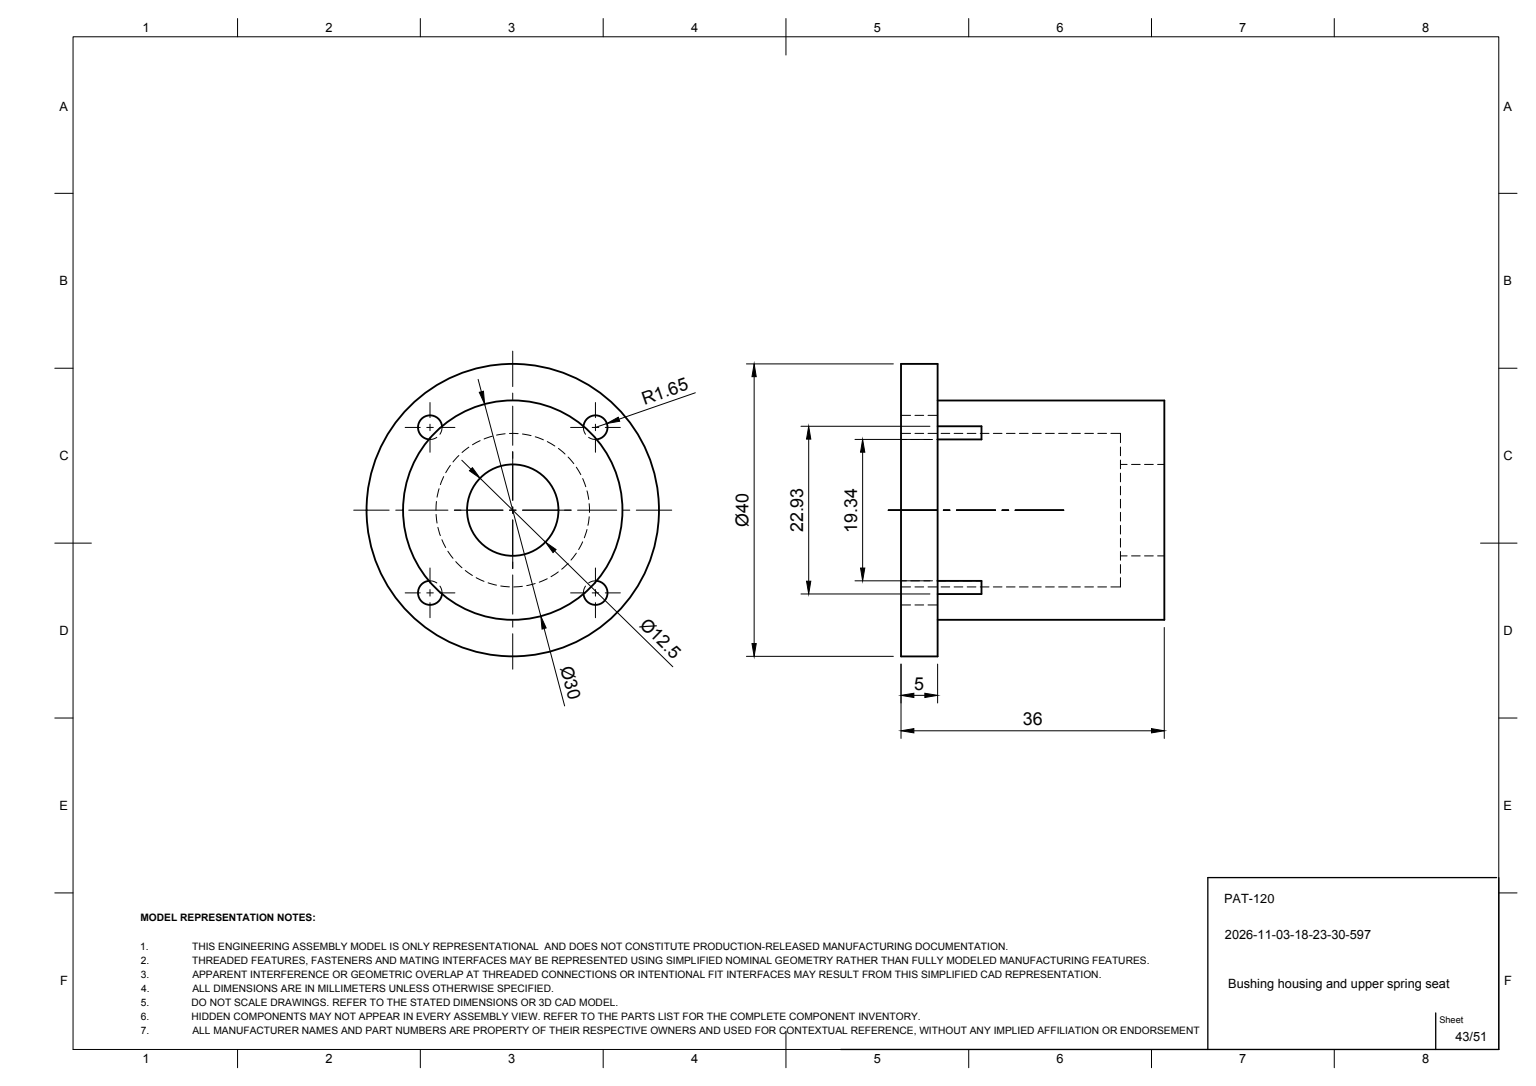
ISO-10303-21;
HEADER;
/* Generated by software containing ST-Developer
 * from STEP Tools, Inc. (www.steptools.com) 
 */

FILE_DESCRIPTION(
/* description */ ('Vibration shaker table dummy'),
/* implementation_level */ '2;1');

FILE_NAME(
/* name */ 'Bushing housing and upper spring seat.step',
/* time_stamp */ '2026-10-27T10:55:14-07:00',
/* author */ (''),
/* organization */ (''),
/* preprocessor_version */ 'ST-DEVELOPER v20.2',
/* originating_system */ 'Autodesk Translation Framework v15.17.0.0',
/* authorisation */ '');

FILE_SCHEMA (('AUTOMOTIVE_DESIGN { 1 0 10303 214 3 1 1 }'));
ENDSEC;

DATA;
#10=MECHANICAL_DESIGN_GEOMETRIC_PRESENTATION_REPRESENTATION('',(#724),#22394);
#632=SHAPE_REPRESENTATION_RELATIONSHIP('SRR','None',#22679,#678);
#678=ADVANCED_BREP_SHAPE_REPRESENTATION('',(#768),#22385);
#724=STYLED_ITEM('',(#22961),#768);
#768=MANIFOLD_SOLID_BREP('Body1',#9244);
#1007=FACE_BOUND('',#2465,.T.);
#1008=FACE_BOUND('',#2467,.T.);
#1009=FACE_BOUND('',#2471,.T.);
#1010=FACE_BOUND('',#2472,.T.);
#1011=FACE_BOUND('',#2473,.T.);
#1012=FACE_BOUND('',#2474,.T.);
#1013=FACE_BOUND('',#2475,.T.);
#1014=FACE_BOUND('',#2477,.T.);
#1278=PLANE('',#10518);
#1279=PLANE('',#10525);
#1280=PLANE('',#10532);
#1281=PLANE('',#10539);
#1282=PLANE('',#10556);
#1283=PLANE('',#10558);
#1284=PLANE('',#10564);
#1285=PLANE('',#10565);
#1724=FACE_OUTER_BOUND('',#2454,.T.);
#1725=FACE_OUTER_BOUND('',#2455,.T.);
#1726=FACE_OUTER_BOUND('',#2456,.T.);
#1727=FACE_OUTER_BOUND('',#2457,.T.);
#1728=FACE_OUTER_BOUND('',#2458,.T.);
#1729=FACE_OUTER_BOUND('',#2459,.T.);
#1730=FACE_OUTER_BOUND('',#2460,.T.);
#1731=FACE_OUTER_BOUND('',#2461,.T.);
#1732=FACE_OUTER_BOUND('',#2462,.T.);
#1733=FACE_OUTER_BOUND('',#2463,.T.);
#1734=FACE_OUTER_BOUND('',#2464,.T.);
#1735=FACE_OUTER_BOUND('',#2466,.T.);
#1736=FACE_OUTER_BOUND('',#2468,.T.);
#1737=FACE_OUTER_BOUND('',#2469,.T.);
#1738=FACE_OUTER_BOUND('',#2470,.T.);
#1739=FACE_OUTER_BOUND('',#2476,.T.);
#2454=EDGE_LOOP('',(#7926,#7927));
#2455=EDGE_LOOP('',(#7928,#7929,#7930,#7931,#7932,#7933,#7934,#7935));
#2456=EDGE_LOOP('',(#7936,#7937));
#2457=EDGE_LOOP('',(#7938,#7939,#7940,#7941,#7942,#7943,#7944,#7945));
#2458=EDGE_LOOP('',(#7946,#7947,#7948));
#2459=EDGE_LOOP('',(#7949,#7950,#7951,#7952,#7953,#7954,#7955,#7956));
#2460=EDGE_LOOP('',(#7957,#7958,#7959));
#2461=EDGE_LOOP('',(#7960,#7961,#7962,#7963,#7964,#7965,#7966,#7967));
#2462=EDGE_LOOP('',(#7968,#7969,#7970,#7971,#7972,#7973,#7974,#7975,#7976,
#7977,#7978,#7979,#7980,#7981,#7982,#7983,#7984,#7985,#7986,#7987));
#2463=EDGE_LOOP('',(#7988,#7989,#7990,#7991));
#2464=EDGE_LOOP('',(#7992));
#2465=EDGE_LOOP('',(#7993));
#2466=EDGE_LOOP('',(#7994));
#2467=EDGE_LOOP('',(#7995,#7996,#7997,#7998,#7999,#8000,#8001,#8002,#8003,
#8004,#8005));
#2468=EDGE_LOOP('',(#8006,#8007,#8008,#8009));
#2469=EDGE_LOOP('',(#8010,#8011,#8012,#8013));
#2470=EDGE_LOOP('',(#8014));
#2471=EDGE_LOOP('',(#8015));
#2472=EDGE_LOOP('',(#8016));
#2473=EDGE_LOOP('',(#8017));
#2474=EDGE_LOOP('',(#8018));
#2475=EDGE_LOOP('',(#8019));
#2476=EDGE_LOOP('',(#8020));
#2477=EDGE_LOOP('',(#8021));
#3121=LINE('',#21556,#3740);
#3122=LINE('',#21560,#3741);
#3123=LINE('',#21564,#3742);
#3124=LINE('',#21572,#3743);
#3125=LINE('',#21576,#3744);
#3126=LINE('',#21580,#3745);
#3127=LINE('',#21590,#3746);
#3128=LINE('',#21593,#3747);
#3129=LINE('',#21595,#3748);
#3130=LINE('',#21606,#3749);
#3131=LINE('',#21609,#3750);
#3132=LINE('',#21611,#3751);
#3133=LINE('',#21617,#3752);
#3134=LINE('',#21627,#3753);
#3135=LINE('',#21638,#3754);
#3136=LINE('',#21641,#3755);
#3740=VECTOR('',#12973,1.);
#3741=VECTOR('',#12976,0.165);
#3742=VECTOR('',#12981,1.);
#3743=VECTOR('',#12990,1.);
#3744=VECTOR('',#12993,0.165);
#3745=VECTOR('',#12998,1.);
#3746=VECTOR('',#13009,1.);
#3747=VECTOR('',#13012,1.);
#3748=VECTOR('',#13013,0.165);
#3749=VECTOR('',#13026,1.);
#3750=VECTOR('',#13029,1.);
#3751=VECTOR('',#13030,0.165);
#3752=VECTOR('',#13037,1.5);
#3753=VECTOR('',#13052,1.05);
#3754=VECTOR('',#13067,2.);
#3755=VECTOR('',#13070,0.625);
#4197=CIRCLE('',#10519,1.5);
#4198=CIRCLE('',#10520,0.165);
#4199=CIRCLE('',#10522,0.165);
#4200=CIRCLE('',#10523,0.165);
#4201=CIRCLE('',#10524,0.165);
#4202=CIRCLE('',#10526,1.5);
#4203=CIRCLE('',#10527,0.165);
#4204=CIRCLE('',#10529,0.165);
#4205=CIRCLE('',#10530,0.165);
#4206=CIRCLE('',#10531,0.165);
#4207=CIRCLE('',#10533,1.5);
#4208=CIRCLE('',#10534,0.165);
#4209=CIRCLE('',#10535,0.165);
#4210=CIRCLE('',#10537,0.165);
#4211=CIRCLE('',#10538,0.165);
#4212=CIRCLE('',#10540,1.5);
#4213=CIRCLE('',#10541,0.165);
#4214=CIRCLE('',#10542,0.165);
#4215=CIRCLE('',#10544,0.165);
#4216=CIRCLE('',#10545,0.165);
#4217=CIRCLE('',#10547,1.5);
#4218=CIRCLE('',#10548,1.5);
#4219=CIRCLE('',#10549,1.5);
#4220=CIRCLE('',#10550,1.5);
#4221=CIRCLE('',#10551,1.5);
#4222=CIRCLE('',#10552,1.5);
#4223=CIRCLE('',#10554,1.05);
#4224=CIRCLE('',#10555,1.05);
#4225=CIRCLE('',#10557,0.625);
#4226=CIRCLE('',#10559,2.);
#4227=CIRCLE('',#10561,2.);
#4228=CIRCLE('',#10563,0.625);
#4924=VERTEX_POINT('',#21550);
#4925=VERTEX_POINT('',#21551);
#4926=VERTEX_POINT('',#21555);
#4927=VERTEX_POINT('',#21557);
#4928=VERTEX_POINT('',#21559);
#4929=VERTEX_POINT('',#21562);
#4930=VERTEX_POINT('',#21566);
#4931=VERTEX_POINT('',#21567);
#4932=VERTEX_POINT('',#21571);
#4933=VERTEX_POINT('',#21573);
#4934=VERTEX_POINT('',#21575);
#4935=VERTEX_POINT('',#21578);
#4936=VERTEX_POINT('',#21582);
#4937=VERTEX_POINT('',#21583);
#4938=VERTEX_POINT('',#21585);
#4939=VERTEX_POINT('',#21589);
#4940=VERTEX_POINT('',#21591);
#4941=VERTEX_POINT('',#21594);
#4942=VERTEX_POINT('',#21598);
#4943=VERTEX_POINT('',#21599);
#4944=VERTEX_POINT('',#21601);
#4945=VERTEX_POINT('',#21605);
#4946=VERTEX_POINT('',#21607);
#4947=VERTEX_POINT('',#21610);
#4948=VERTEX_POINT('',#21614);
#4949=VERTEX_POINT('',#21616);
#4950=VERTEX_POINT('',#21624);
#4951=VERTEX_POINT('',#21626);
#4952=VERTEX_POINT('',#21630);
#4953=VERTEX_POINT('',#21633);
#4954=VERTEX_POINT('',#21636);
#4955=VERTEX_POINT('',#21640);
#5956=EDGE_CURVE('',#4924,#4925,#4197,.T.);
#5957=EDGE_CURVE('',#4924,#4925,#4198,.T.);
#5958=EDGE_CURVE('',#4926,#4924,#3121,.T.);
#5959=EDGE_CURVE('',#4927,#4926,#4199,.T.);
#5960=EDGE_CURVE('',#4927,#4928,#3122,.T.);
#5961=EDGE_CURVE('',#4928,#4928,#4200,.T.);
#5962=EDGE_CURVE('',#4929,#4927,#4201,.T.);
#5963=EDGE_CURVE('',#4925,#4929,#3123,.T.);
#5964=EDGE_CURVE('',#4930,#4931,#4202,.T.);
#5965=EDGE_CURVE('',#4930,#4931,#4203,.T.);
#5966=EDGE_CURVE('',#4932,#4930,#3124,.T.);
#5967=EDGE_CURVE('',#4933,#4932,#4204,.T.);
#5968=EDGE_CURVE('',#4933,#4934,#3125,.T.);
#5969=EDGE_CURVE('',#4934,#4934,#4205,.T.);
#5970=EDGE_CURVE('',#4935,#4933,#4206,.T.);
#5971=EDGE_CURVE('',#4931,#4935,#3126,.T.);
#5972=EDGE_CURVE('',#4936,#4937,#4207,.T.);
#5973=EDGE_CURVE('',#4936,#4938,#4208,.T.);
#5974=EDGE_CURVE('',#4938,#4937,#4209,.T.);
#5975=EDGE_CURVE('',#4939,#4936,#3127,.T.);
#5976=EDGE_CURVE('',#4940,#4939,#4210,.T.);
#5977=EDGE_CURVE('',#4937,#4940,#3128,.T.);
#5978=EDGE_CURVE('',#4938,#4941,#3129,.T.);
#5979=EDGE_CURVE('',#4941,#4941,#4211,.T.);
#5980=EDGE_CURVE('',#4942,#4943,#4212,.T.);
#5981=EDGE_CURVE('',#4942,#4944,#4213,.T.);
#5982=EDGE_CURVE('',#4944,#4943,#4214,.T.);
#5983=EDGE_CURVE('',#4945,#4942,#3130,.T.);
#5984=EDGE_CURVE('',#4946,#4945,#4215,.T.);
#5985=EDGE_CURVE('',#4943,#4946,#3131,.T.);
#5986=EDGE_CURVE('',#4944,#4947,#3132,.T.);
#5987=EDGE_CURVE('',#4947,#4947,#4216,.T.);
#5988=EDGE_CURVE('',#4929,#4948,#4217,.T.);
#5989=EDGE_CURVE('',#4948,#4949,#3133,.T.);
#5990=EDGE_CURVE('',#4949,#4949,#4218,.T.);
#5991=EDGE_CURVE('',#4948,#4932,#4219,.T.);
#5992=EDGE_CURVE('',#4935,#4939,#4220,.T.);
#5993=EDGE_CURVE('',#4940,#4945,#4221,.T.);
#5994=EDGE_CURVE('',#4946,#4926,#4222,.T.);
#5995=EDGE_CURVE('',#4950,#4950,#4223,.T.);
#5996=EDGE_CURVE('',#4950,#4951,#3134,.T.);
#5997=EDGE_CURVE('',#4951,#4951,#4224,.T.);
#5998=EDGE_CURVE('',#4952,#4952,#4225,.T.);
#5999=EDGE_CURVE('',#4953,#4953,#4226,.T.);
#6000=EDGE_CURVE('',#4954,#4954,#4227,.T.);
#6001=EDGE_CURVE('',#4954,#4953,#3135,.T.);
#6002=EDGE_CURVE('',#4952,#4955,#3136,.T.);
#6003=EDGE_CURVE('',#4955,#4955,#4228,.T.);
#7926=ORIENTED_EDGE('',*,*,#5956,.F.);
#7927=ORIENTED_EDGE('',*,*,#5957,.T.);
#7928=ORIENTED_EDGE('',*,*,#5958,.F.);
#7929=ORIENTED_EDGE('',*,*,#5959,.F.);
#7930=ORIENTED_EDGE('',*,*,#5960,.T.);
#7931=ORIENTED_EDGE('',*,*,#5961,.F.);
#7932=ORIENTED_EDGE('',*,*,#5960,.F.);
#7933=ORIENTED_EDGE('',*,*,#5962,.F.);
#7934=ORIENTED_EDGE('',*,*,#5963,.F.);
#7935=ORIENTED_EDGE('',*,*,#5957,.F.);
#7936=ORIENTED_EDGE('',*,*,#5964,.F.);
#7937=ORIENTED_EDGE('',*,*,#5965,.T.);
#7938=ORIENTED_EDGE('',*,*,#5966,.F.);
#7939=ORIENTED_EDGE('',*,*,#5967,.F.);
#7940=ORIENTED_EDGE('',*,*,#5968,.T.);
#7941=ORIENTED_EDGE('',*,*,#5969,.F.);
#7942=ORIENTED_EDGE('',*,*,#5968,.F.);
#7943=ORIENTED_EDGE('',*,*,#5970,.F.);
#7944=ORIENTED_EDGE('',*,*,#5971,.F.);
#7945=ORIENTED_EDGE('',*,*,#5965,.F.);
#7946=ORIENTED_EDGE('',*,*,#5972,.F.);
#7947=ORIENTED_EDGE('',*,*,#5973,.T.);
#7948=ORIENTED_EDGE('',*,*,#5974,.T.);
#7949=ORIENTED_EDGE('',*,*,#5975,.F.);
#7950=ORIENTED_EDGE('',*,*,#5976,.F.);
#7951=ORIENTED_EDGE('',*,*,#5977,.F.);
#7952=ORIENTED_EDGE('',*,*,#5974,.F.);
#7953=ORIENTED_EDGE('',*,*,#5978,.T.);
#7954=ORIENTED_EDGE('',*,*,#5979,.F.);
#7955=ORIENTED_EDGE('',*,*,#5978,.F.);
#7956=ORIENTED_EDGE('',*,*,#5973,.F.);
#7957=ORIENTED_EDGE('',*,*,#5980,.F.);
#7958=ORIENTED_EDGE('',*,*,#5981,.T.);
#7959=ORIENTED_EDGE('',*,*,#5982,.T.);
#7960=ORIENTED_EDGE('',*,*,#5983,.F.);
#7961=ORIENTED_EDGE('',*,*,#5984,.F.);
#7962=ORIENTED_EDGE('',*,*,#5985,.F.);
#7963=ORIENTED_EDGE('',*,*,#5982,.F.);
#7964=ORIENTED_EDGE('',*,*,#5986,.T.);
#7965=ORIENTED_EDGE('',*,*,#5987,.F.);
#7966=ORIENTED_EDGE('',*,*,#5986,.F.);
#7967=ORIENTED_EDGE('',*,*,#5981,.F.);
#7968=ORIENTED_EDGE('',*,*,#5958,.T.);
#7969=ORIENTED_EDGE('',*,*,#5956,.T.);
#7970=ORIENTED_EDGE('',*,*,#5963,.T.);
#7971=ORIENTED_EDGE('',*,*,#5988,.T.);
#7972=ORIENTED_EDGE('',*,*,#5989,.T.);
#7973=ORIENTED_EDGE('',*,*,#5990,.T.);
#7974=ORIENTED_EDGE('',*,*,#5989,.F.);
#7975=ORIENTED_EDGE('',*,*,#5991,.T.);
#7976=ORIENTED_EDGE('',*,*,#5966,.T.);
#7977=ORIENTED_EDGE('',*,*,#5964,.T.);
#7978=ORIENTED_EDGE('',*,*,#5971,.T.);
#7979=ORIENTED_EDGE('',*,*,#5992,.T.);
#7980=ORIENTED_EDGE('',*,*,#5975,.T.);
#7981=ORIENTED_EDGE('',*,*,#5972,.T.);
#7982=ORIENTED_EDGE('',*,*,#5977,.T.);
#7983=ORIENTED_EDGE('',*,*,#5993,.T.);
#7984=ORIENTED_EDGE('',*,*,#5983,.T.);
#7985=ORIENTED_EDGE('',*,*,#5980,.T.);
#7986=ORIENTED_EDGE('',*,*,#5985,.T.);
#7987=ORIENTED_EDGE('',*,*,#5994,.T.);
#7988=ORIENTED_EDGE('',*,*,#5995,.F.);
#7989=ORIENTED_EDGE('',*,*,#5996,.T.);
#7990=ORIENTED_EDGE('',*,*,#5997,.F.);
#7991=ORIENTED_EDGE('',*,*,#5996,.F.);
#7992=ORIENTED_EDGE('',*,*,#5995,.T.);
#7993=ORIENTED_EDGE('',*,*,#5998,.F.);
#7994=ORIENTED_EDGE('',*,*,#5999,.F.);
#7995=ORIENTED_EDGE('',*,*,#5962,.T.);
#7996=ORIENTED_EDGE('',*,*,#5959,.T.);
#7997=ORIENTED_EDGE('',*,*,#5994,.F.);
#7998=ORIENTED_EDGE('',*,*,#5984,.T.);
#7999=ORIENTED_EDGE('',*,*,#5993,.F.);
#8000=ORIENTED_EDGE('',*,*,#5976,.T.);
#8001=ORIENTED_EDGE('',*,*,#5992,.F.);
#8002=ORIENTED_EDGE('',*,*,#5970,.T.);
#8003=ORIENTED_EDGE('',*,*,#5967,.T.);
#8004=ORIENTED_EDGE('',*,*,#5991,.F.);
#8005=ORIENTED_EDGE('',*,*,#5988,.F.);
#8006=ORIENTED_EDGE('',*,*,#6000,.F.);
#8007=ORIENTED_EDGE('',*,*,#6001,.T.);
#8008=ORIENTED_EDGE('',*,*,#5999,.T.);
#8009=ORIENTED_EDGE('',*,*,#6001,.F.);
#8010=ORIENTED_EDGE('',*,*,#5998,.T.);
#8011=ORIENTED_EDGE('',*,*,#6002,.T.);
#8012=ORIENTED_EDGE('',*,*,#6003,.T.);
#8013=ORIENTED_EDGE('',*,*,#6002,.F.);
#8014=ORIENTED_EDGE('',*,*,#6000,.T.);
#8015=ORIENTED_EDGE('',*,*,#5997,.T.);
#8016=ORIENTED_EDGE('',*,*,#5987,.T.);
#8017=ORIENTED_EDGE('',*,*,#5979,.T.);
#8018=ORIENTED_EDGE('',*,*,#5969,.T.);
#8019=ORIENTED_EDGE('',*,*,#5961,.T.);
#8020=ORIENTED_EDGE('',*,*,#5990,.F.);
#8021=ORIENTED_EDGE('',*,*,#6003,.F.);
#8658=CYLINDRICAL_SURFACE('',#10521,0.165);
#8659=CYLINDRICAL_SURFACE('',#10528,0.165);
#8660=CYLINDRICAL_SURFACE('',#10536,0.165);
#8661=CYLINDRICAL_SURFACE('',#10543,0.165);
#8662=CYLINDRICAL_SURFACE('',#10546,1.5);
#8663=CYLINDRICAL_SURFACE('',#10553,1.05);
#8664=CYLINDRICAL_SURFACE('',#10560,2.);
#8665=CYLINDRICAL_SURFACE('',#10562,0.625);
#9089=ADVANCED_FACE('',(#1724),#1278,.T.);
#9090=ADVANCED_FACE('',(#1725),#8658,.F.);
#9091=ADVANCED_FACE('',(#1726),#1279,.T.);
#9092=ADVANCED_FACE('',(#1727),#8659,.F.);
#9093=ADVANCED_FACE('',(#1728),#1280,.T.);
#9094=ADVANCED_FACE('',(#1729),#8660,.F.);
#9095=ADVANCED_FACE('',(#1730),#1281,.T.);
#9096=ADVANCED_FACE('',(#1731),#8661,.F.);
#9097=ADVANCED_FACE('',(#1732),#8662,.T.);
#9098=ADVANCED_FACE('',(#1733),#8663,.F.);
#9099=ADVANCED_FACE('',(#1734,#1007),#1282,.T.);
#9100=ADVANCED_FACE('',(#1735,#1008),#1283,.F.);
#9101=ADVANCED_FACE('',(#1736),#8664,.T.);
#9102=ADVANCED_FACE('',(#1737),#8665,.F.);
#9103=ADVANCED_FACE('',(#1738,#1009,#1010,#1011,#1012,#1013),#1284,.T.);
#9104=ADVANCED_FACE('',(#1739,#1014),#1285,.F.);
#9244=CLOSED_SHELL('',(#9089,#9090,#9091,#9092,#9093,#9094,#9095,#9096,
#9097,#9098,#9099,#9100,#9101,#9102,#9103,#9104));
#10517=AXIS2_PLACEMENT_3D('',#21548,#12963,#12964);
#10518=AXIS2_PLACEMENT_3D('',#21549,#12965,#12966);
#10519=AXIS2_PLACEMENT_3D('',#21552,#12967,#12968);
#10520=AXIS2_PLACEMENT_3D('',#21553,#12969,#12970);
#10521=AXIS2_PLACEMENT_3D('',#21554,#12971,#12972);
#10522=AXIS2_PLACEMENT_3D('',#21558,#12974,#12975);
#10523=AXIS2_PLACEMENT_3D('',#21561,#12977,#12978);
#10524=AXIS2_PLACEMENT_3D('',#21563,#12979,#12980);
#10525=AXIS2_PLACEMENT_3D('',#21565,#12982,#12983);
#10526=AXIS2_PLACEMENT_3D('',#21568,#12984,#12985);
#10527=AXIS2_PLACEMENT_3D('',#21569,#12986,#12987);
#10528=AXIS2_PLACEMENT_3D('',#21570,#12988,#12989);
#10529=AXIS2_PLACEMENT_3D('',#21574,#12991,#12992);
#10530=AXIS2_PLACEMENT_3D('',#21577,#12994,#12995);
#10531=AXIS2_PLACEMENT_3D('',#21579,#12996,#12997);
#10532=AXIS2_PLACEMENT_3D('',#21581,#12999,#13000);
#10533=AXIS2_PLACEMENT_3D('',#21584,#13001,#13002);
#10534=AXIS2_PLACEMENT_3D('',#21586,#13003,#13004);
#10535=AXIS2_PLACEMENT_3D('',#21587,#13005,#13006);
#10536=AXIS2_PLACEMENT_3D('',#21588,#13007,#13008);
#10537=AXIS2_PLACEMENT_3D('',#21592,#13010,#13011);
#10538=AXIS2_PLACEMENT_3D('',#21596,#13014,#13015);
#10539=AXIS2_PLACEMENT_3D('',#21597,#13016,#13017);
#10540=AXIS2_PLACEMENT_3D('',#21600,#13018,#13019);
#10541=AXIS2_PLACEMENT_3D('',#21602,#13020,#13021);
#10542=AXIS2_PLACEMENT_3D('',#21603,#13022,#13023);
#10543=AXIS2_PLACEMENT_3D('',#21604,#13024,#13025);
#10544=AXIS2_PLACEMENT_3D('',#21608,#13027,#13028);
#10545=AXIS2_PLACEMENT_3D('',#21612,#13031,#13032);
#10546=AXIS2_PLACEMENT_3D('',#21613,#13033,#13034);
#10547=AXIS2_PLACEMENT_3D('',#21615,#13035,#13036);
#10548=AXIS2_PLACEMENT_3D('',#21618,#13038,#13039);
#10549=AXIS2_PLACEMENT_3D('',#21619,#13040,#13041);
#10550=AXIS2_PLACEMENT_3D('',#21620,#13042,#13043);
#10551=AXIS2_PLACEMENT_3D('',#21621,#13044,#13045);
#10552=AXIS2_PLACEMENT_3D('',#21622,#13046,#13047);
#10553=AXIS2_PLACEMENT_3D('',#21623,#13048,#13049);
#10554=AXIS2_PLACEMENT_3D('',#21625,#13050,#13051);
#10555=AXIS2_PLACEMENT_3D('',#21628,#13053,#13054);
#10556=AXIS2_PLACEMENT_3D('',#21629,#13055,#13056);
#10557=AXIS2_PLACEMENT_3D('',#21631,#13057,#13058);
#10558=AXIS2_PLACEMENT_3D('',#21632,#13059,#13060);
#10559=AXIS2_PLACEMENT_3D('',#21634,#13061,#13062);
#10560=AXIS2_PLACEMENT_3D('',#21635,#13063,#13064);
#10561=AXIS2_PLACEMENT_3D('',#21637,#13065,#13066);
#10562=AXIS2_PLACEMENT_3D('',#21639,#13068,#13069);
#10563=AXIS2_PLACEMENT_3D('',#21642,#13071,#13072);
#10564=AXIS2_PLACEMENT_3D('',#21643,#13073,#13074);
#10565=AXIS2_PLACEMENT_3D('',#21644,#13075,#13076);
#12963=DIRECTION('axis',(0.,0.,1.));
#12964=DIRECTION('refdir',(1.,0.,0.));
#12965=DIRECTION('center_axis',(0.,0.,1.));
#12966=DIRECTION('ref_axis',(1.,0.,0.));
#12967=DIRECTION('center_axis',(0.,0.,-1.));
#12968=DIRECTION('ref_axis',(1.,0.,0.));
#12969=DIRECTION('center_axis',(0.,0.,1.));
#12970=DIRECTION('ref_axis',(1.,0.,0.));
#12971=DIRECTION('center_axis',(0.,0.,1.));
#12972=DIRECTION('ref_axis',(1.,0.,0.));
#12973=DIRECTION('',(0.,0.,-1.));
#12974=DIRECTION('center_axis',(0.,0.,1.));
#12975=DIRECTION('ref_axis',(1.,0.,0.));
#12976=DIRECTION('',(0.,0.,1.));
#12977=DIRECTION('center_axis',(0.,0.,-1.));
#12978=DIRECTION('ref_axis',(1.,0.,0.));
#12979=DIRECTION('center_axis',(0.,0.,1.));
#12980=DIRECTION('ref_axis',(1.,0.,0.));
#12981=DIRECTION('',(0.,0.,1.));
#12982=DIRECTION('center_axis',(0.,0.,1.));
#12983=DIRECTION('ref_axis',(1.,0.,0.));
#12984=DIRECTION('center_axis',(0.,0.,-1.));
#12985=DIRECTION('ref_axis',(1.,0.,0.));
#12986=DIRECTION('center_axis',(0.,0.,1.));
#12987=DIRECTION('ref_axis',(1.,0.,0.));
#12988=DIRECTION('center_axis',(0.,0.,1.));
#12989=DIRECTION('ref_axis',(1.,0.,0.));
#12990=DIRECTION('',(0.,0.,-1.));
#12991=DIRECTION('center_axis',(0.,0.,1.));
#12992=DIRECTION('ref_axis',(1.,0.,0.));
#12993=DIRECTION('',(0.,0.,1.));
#12994=DIRECTION('center_axis',(0.,0.,-1.));
#12995=DIRECTION('ref_axis',(1.,0.,0.));
#12996=DIRECTION('center_axis',(0.,0.,1.));
#12997=DIRECTION('ref_axis',(1.,0.,0.));
#12998=DIRECTION('',(0.,0.,1.));
#12999=DIRECTION('center_axis',(0.,0.,1.));
#13000=DIRECTION('ref_axis',(1.,0.,0.));
#13001=DIRECTION('center_axis',(0.,0.,-1.));
#13002=DIRECTION('ref_axis',(1.,0.,0.));
#13003=DIRECTION('center_axis',(0.,0.,1.));
#13004=DIRECTION('ref_axis',(1.,0.,0.));
#13005=DIRECTION('center_axis',(0.,0.,1.));
#13006=DIRECTION('ref_axis',(1.,0.,0.));
#13007=DIRECTION('center_axis',(0.,0.,1.));
#13008=DIRECTION('ref_axis',(1.,0.,0.));
#13009=DIRECTION('',(0.,0.,-1.));
#13010=DIRECTION('center_axis',(0.,0.,1.));
#13011=DIRECTION('ref_axis',(1.,0.,0.));
#13012=DIRECTION('',(0.,0.,1.));
#13013=DIRECTION('',(0.,0.,1.));
#13014=DIRECTION('center_axis',(0.,0.,-1.));
#13015=DIRECTION('ref_axis',(1.,0.,0.));
#13016=DIRECTION('center_axis',(0.,0.,1.));
#13017=DIRECTION('ref_axis',(1.,0.,0.));
#13018=DIRECTION('center_axis',(0.,0.,-1.));
#13019=DIRECTION('ref_axis',(1.,0.,0.));
#13020=DIRECTION('center_axis',(0.,0.,1.));
#13021=DIRECTION('ref_axis',(1.,0.,0.));
#13022=DIRECTION('center_axis',(0.,0.,1.));
#13023=DIRECTION('ref_axis',(1.,0.,0.));
#13024=DIRECTION('center_axis',(0.,0.,1.));
#13025=DIRECTION('ref_axis',(1.,0.,0.));
#13026=DIRECTION('',(0.,0.,-1.));
#13027=DIRECTION('center_axis',(0.,0.,1.));
#13028=DIRECTION('ref_axis',(1.,0.,0.));
#13029=DIRECTION('',(0.,0.,1.));
#13030=DIRECTION('',(0.,0.,1.));
#13031=DIRECTION('center_axis',(0.,0.,-1.));
#13032=DIRECTION('ref_axis',(1.,0.,0.));
#13033=DIRECTION('center_axis',(0.,0.,1.));
#13034=DIRECTION('ref_axis',(1.,0.,0.));
#13035=DIRECTION('center_axis',(0.,0.,-1.));
#13036=DIRECTION('ref_axis',(1.,0.,0.));
#13037=DIRECTION('',(0.,0.,-1.));
#13038=DIRECTION('center_axis',(0.,0.,1.));
#13039=DIRECTION('ref_axis',(1.,0.,0.));
#13040=DIRECTION('center_axis',(0.,0.,-1.));
#13041=DIRECTION('ref_axis',(1.,0.,0.));
#13042=DIRECTION('center_axis',(0.,0.,-1.));
#13043=DIRECTION('ref_axis',(1.,0.,0.));
#13044=DIRECTION('center_axis',(0.,0.,-1.));
#13045=DIRECTION('ref_axis',(1.,0.,0.));
#13046=DIRECTION('center_axis',(0.,0.,-1.));
#13047=DIRECTION('ref_axis',(1.,0.,0.));
#13048=DIRECTION('center_axis',(0.,0.,1.));
#13049=DIRECTION('ref_axis',(1.,0.,0.));
#13050=DIRECTION('center_axis',(0.,0.,1.));
#13051=DIRECTION('ref_axis',(1.,0.,0.));
#13052=DIRECTION('',(0.,0.,1.));
#13053=DIRECTION('center_axis',(0.,0.,-1.));
#13054=DIRECTION('ref_axis',(1.,0.,0.));
#13055=DIRECTION('center_axis',(0.,0.,1.));
#13056=DIRECTION('ref_axis',(1.,0.,0.));
#13057=DIRECTION('center_axis',(0.,0.,1.));
#13058=DIRECTION('ref_axis',(1.,0.,0.));
#13059=DIRECTION('center_axis',(0.,0.,1.));
#13060=DIRECTION('ref_axis',(1.,0.,0.));
#13061=DIRECTION('center_axis',(0.,0.,1.));
#13062=DIRECTION('ref_axis',(1.,0.,0.));
#13063=DIRECTION('center_axis',(0.,0.,1.));
#13064=DIRECTION('ref_axis',(1.,0.,0.));
#13065=DIRECTION('center_axis',(0.,0.,1.));
#13066=DIRECTION('ref_axis',(1.,0.,0.));
#13067=DIRECTION('',(0.,0.,-1.));
#13068=DIRECTION('center_axis',(0.,0.,1.));
#13069=DIRECTION('ref_axis',(1.,0.,0.));
#13070=DIRECTION('',(0.,0.,-1.));
#13071=DIRECTION('center_axis',(0.,0.,-1.));
#13072=DIRECTION('ref_axis',(1.,0.,0.));
#13073=DIRECTION('center_axis',(0.,0.,1.));
#13074=DIRECTION('ref_axis',(1.,0.,0.));
#13075=DIRECTION('center_axis',(0.,0.,1.));
#13076=DIRECTION('ref_axis',(1.,0.,0.));
#21548=CARTESIAN_POINT('',(0.,0.,0.));
#21549=CARTESIAN_POINT('Origin',(-7.13137084989848,-5.13137084989848,14.));
#21550=CARTESIAN_POINT('',(-6.96707794165985,-5.14662995545858,14.));
#21551=CARTESIAN_POINT('',(-7.14662995545858,-4.96707794165985,14.));
#21552=CARTESIAN_POINT('Origin',(-6.,-4.,14.));
#21553=CARTESIAN_POINT('Origin',(-7.13137084989848,-5.13137084989848,14.));
#21554=CARTESIAN_POINT('Origin',(-7.13137084989848,-5.13137084989848,14.));
#21555=CARTESIAN_POINT('',(-6.96707794165985,-5.14662995545858,14.6));
#21556=CARTESIAN_POINT('',(-6.96707794165985,-5.14662995545858,14.));
#21557=CARTESIAN_POINT('',(-7.29637084989848,-5.13137084989848,14.6));
#21558=CARTESIAN_POINT('Origin',(-7.13137084989848,-5.13137084989848,14.6));
#21559=CARTESIAN_POINT('',(-7.29637084989848,-5.13137084989848,15.1));
#21560=CARTESIAN_POINT('',(-7.29637084989848,-5.13137084989848,14.));
#21561=CARTESIAN_POINT('Origin',(-7.13137084989848,-5.13137084989848,15.1));
#21562=CARTESIAN_POINT('',(-7.14662995545858,-4.96707794165985,14.6));
#21563=CARTESIAN_POINT('Origin',(-7.13137084989848,-5.13137084989848,14.6));
#21564=CARTESIAN_POINT('',(-7.14662995545858,-4.96707794165985,14.));
#21565=CARTESIAN_POINT('Origin',(-7.13137084989848,-2.86862915010152,14.));
#21566=CARTESIAN_POINT('',(-7.14662995545858,-3.03292205834015,14.));
#21567=CARTESIAN_POINT('',(-6.96707794165985,-2.85337004454142,14.));
#21568=CARTESIAN_POINT('Origin',(-6.,-4.,14.));
#21569=CARTESIAN_POINT('Origin',(-7.13137084989848,-2.86862915010152,14.));
#21570=CARTESIAN_POINT('Origin',(-7.13137084989848,-2.86862915010152,14.));
#21571=CARTESIAN_POINT('',(-7.14662995545858,-3.03292205834015,14.6));
#21572=CARTESIAN_POINT('',(-7.14662995545858,-3.03292205834015,14.));
#21573=CARTESIAN_POINT('',(-7.29637084989848,-2.86862915010152,14.6));
#21574=CARTESIAN_POINT('Origin',(-7.13137084989848,-2.86862915010152,14.6));
#21575=CARTESIAN_POINT('',(-7.29637084989848,-2.86862915010152,15.1));
#21576=CARTESIAN_POINT('',(-7.29637084989848,-2.86862915010152,14.));
#21577=CARTESIAN_POINT('Origin',(-7.13137084989848,-2.86862915010152,15.1));
#21578=CARTESIAN_POINT('',(-6.96707794165985,-2.85337004454142,14.6));
#21579=CARTESIAN_POINT('Origin',(-7.13137084989848,-2.86862915010152,14.6));
#21580=CARTESIAN_POINT('',(-6.96707794165985,-2.85337004454142,14.));
#21581=CARTESIAN_POINT('Origin',(-4.86862915010152,-2.86862915010152,14.));
#21582=CARTESIAN_POINT('',(-5.03292205834015,-2.85337004454142,14.));
#21583=CARTESIAN_POINT('',(-4.85337004454142,-3.03292205834015,14.));
#21584=CARTESIAN_POINT('Origin',(-6.,-4.,14.));
#21585=CARTESIAN_POINT('',(-5.03362915010152,-2.86862915010152,14.));
#21586=CARTESIAN_POINT('Origin',(-4.86862915010152,-2.86862915010152,14.));
#21587=CARTESIAN_POINT('Origin',(-4.86862915010152,-2.86862915010152,14.));
#21588=CARTESIAN_POINT('Origin',(-4.86862915010152,-2.86862915010152,14.));
#21589=CARTESIAN_POINT('',(-5.03292205834015,-2.85337004454142,14.6));
#21590=CARTESIAN_POINT('',(-5.03292205834015,-2.85337004454142,14.));
#21591=CARTESIAN_POINT('',(-4.85337004454142,-3.03292205834015,14.6));
#21592=CARTESIAN_POINT('Origin',(-4.86862915010152,-2.86862915010152,14.6));
#21593=CARTESIAN_POINT('',(-4.85337004454142,-3.03292205834015,14.));
#21594=CARTESIAN_POINT('',(-5.03362915010152,-2.86862915010152,15.1));
#21595=CARTESIAN_POINT('',(-5.03362915010152,-2.86862915010152,14.));
#21596=CARTESIAN_POINT('Origin',(-4.86862915010152,-2.86862915010152,15.1));
#21597=CARTESIAN_POINT('Origin',(-4.86862915010152,-5.13137084989848,14.));
#21598=CARTESIAN_POINT('',(-4.85337004454142,-4.96707794165985,14.));
#21599=CARTESIAN_POINT('',(-5.03292205834015,-5.14662995545858,14.));
#21600=CARTESIAN_POINT('Origin',(-6.,-4.,14.));
#21601=CARTESIAN_POINT('',(-5.03362915010152,-5.13137084989848,14.));
#21602=CARTESIAN_POINT('Origin',(-4.86862915010152,-5.13137084989848,14.));
#21603=CARTESIAN_POINT('Origin',(-4.86862915010152,-5.13137084989848,14.));
#21604=CARTESIAN_POINT('Origin',(-4.86862915010152,-5.13137084989848,14.));
#21605=CARTESIAN_POINT('',(-4.85337004454142,-4.96707794165985,14.6));
#21606=CARTESIAN_POINT('',(-4.85337004454142,-4.96707794165985,14.));
#21607=CARTESIAN_POINT('',(-5.03292205834015,-5.14662995545858,14.6));
#21608=CARTESIAN_POINT('Origin',(-4.86862915010152,-5.13137084989848,14.6));
#21609=CARTESIAN_POINT('',(-5.03292205834015,-5.14662995545858,14.));
#21610=CARTESIAN_POINT('',(-5.03362915010152,-5.13137084989848,15.1));
#21611=CARTESIAN_POINT('',(-5.03362915010152,-5.13137084989848,14.));
#21612=CARTESIAN_POINT('Origin',(-4.86862915010152,-5.13137084989848,15.1));
#21613=CARTESIAN_POINT('Origin',(-6.,-4.,11.5));
#21614=CARTESIAN_POINT('',(-7.5,-4.,14.6));
#21615=CARTESIAN_POINT('Origin',(-6.,-4.,14.6));
#21616=CARTESIAN_POINT('',(-7.5,-4.,11.5));
#21617=CARTESIAN_POINT('',(-7.5,-4.,11.5));
#21618=CARTESIAN_POINT('Origin',(-6.,-4.,11.5));
#21619=CARTESIAN_POINT('Origin',(-6.,-4.,14.6));
#21620=CARTESIAN_POINT('Origin',(-6.,-4.,14.6));
#21621=CARTESIAN_POINT('Origin',(-6.,-4.,14.6));
#21622=CARTESIAN_POINT('Origin',(-6.,-4.,14.6));
#21623=CARTESIAN_POINT('Origin',(-6.,-4.,12.1));
#21624=CARTESIAN_POINT('',(-7.05,-4.,12.1));
#21625=CARTESIAN_POINT('Origin',(-6.,-4.,12.1));
#21626=CARTESIAN_POINT('',(-7.05,-4.,15.1));
#21627=CARTESIAN_POINT('',(-7.05,-4.,12.1));
#21628=CARTESIAN_POINT('Origin',(-6.,-4.,15.1));
#21629=CARTESIAN_POINT('Origin',(-6.,-4.,12.1));
#21630=CARTESIAN_POINT('',(-6.625,-4.,12.1));
#21631=CARTESIAN_POINT('Origin',(-6.,-4.,12.1));
#21632=CARTESIAN_POINT('Origin',(-6.,-4.,14.6));
#21633=CARTESIAN_POINT('',(-8.,-4.,14.6));
#21634=CARTESIAN_POINT('Origin',(-6.,-4.,14.6));
#21635=CARTESIAN_POINT('Origin',(-6.,-4.,14.6));
#21636=CARTESIAN_POINT('',(-8.,-4.,15.1));
#21637=CARTESIAN_POINT('Origin',(-6.,-4.,15.1));
#21638=CARTESIAN_POINT('',(-8.,-4.,14.6));
#21639=CARTESIAN_POINT('Origin',(-6.,-4.,11.5));
#21640=CARTESIAN_POINT('',(-6.625,-4.,11.5));
#21641=CARTESIAN_POINT('',(-6.625,-4.,11.5));
#21642=CARTESIAN_POINT('Origin',(-6.,-4.,11.5));
#21643=CARTESIAN_POINT('Origin',(-6.,-4.,15.1));
#21644=CARTESIAN_POINT('Origin',(-6.,-4.,11.5));
#22334=UNCERTAINTY_MEASURE_WITH_UNIT(LENGTH_MEASURE(0.001),#22395,
'DISTANCE_ACCURACY_VALUE',
'Maximum model space distance between geometric entities at asserted c
onnectivities');
#22343=UNCERTAINTY_MEASURE_WITH_UNIT(LENGTH_MEASURE(0.001),#22395,
'DISTANCE_ACCURACY_VALUE',
'Maximum model space distance between geometric entities at asserted c
onnectivities');
#22385=(
GEOMETRIC_REPRESENTATION_CONTEXT(3)
GLOBAL_UNCERTAINTY_ASSIGNED_CONTEXT((#22334))
GLOBAL_UNIT_ASSIGNED_CONTEXT((#22395,#22397,#22398))
REPRESENTATION_CONTEXT('','3D')
);
#22394=(
GEOMETRIC_REPRESENTATION_CONTEXT(3)
GLOBAL_UNCERTAINTY_ASSIGNED_CONTEXT((#22343))
GLOBAL_UNIT_ASSIGNED_CONTEXT((#22395,#22397,#22398))
REPRESENTATION_CONTEXT('','3D')
);
#22395=(
LENGTH_UNIT()
NAMED_UNIT(*)
SI_UNIT(.CENTI.,.METRE.)
);
#22397=(
NAMED_UNIT(*)
PLANE_ANGLE_UNIT()
SI_UNIT($,.RADIAN.)
);
#22398=(
NAMED_UNIT(*)
SI_UNIT($,.STERADIAN.)
SOLID_ANGLE_UNIT()
);
#22440=SHAPE_DEFINITION_REPRESENTATION(#22490,#22679);
#22490=PRODUCT_DEFINITION_SHAPE('',$,#22730);
#22679=SHAPE_REPRESENTATION('',(#10517),#22385);
#22688=PRODUCT_DEFINITION_CONTEXT('part definition',#22840,'design');
#22730=PRODUCT_DEFINITION('Bushing housing and upper spring seat',
'Bushing housing and upper spring seat',#22780,#22688);
#22780=PRODUCT_DEFINITION_FORMATION('',$,#22883);
#22840=APPLICATION_CONTEXT(
'Core Data for Automotive Mechanical Design Process');
#22841=PRODUCT_CONTEXT('part definition',#22840,'mechanical');
#22883=PRODUCT('Bushing housing and upper spring seat',
'Bushing housing and upper spring seat',
'Bushing housing and upper spring seat',(#22841));
#22955=COLOUR_RGB('Grey',0.48,0.52,0.57);
#22956=FILL_AREA_STYLE_COLOUR('',#22955);
#22957=FILL_AREA_STYLE('',(#22956));
#22958=SURFACE_STYLE_FILL_AREA(#22957);
#22959=SURFACE_SIDE_STYLE('',(#22958));
#22960=SURFACE_STYLE_USAGE(.BOTH.,#22959);
#22961=PRESENTATION_STYLE_ASSIGNMENT((#22960));
ENDSEC;
END-ISO-10303-21;
